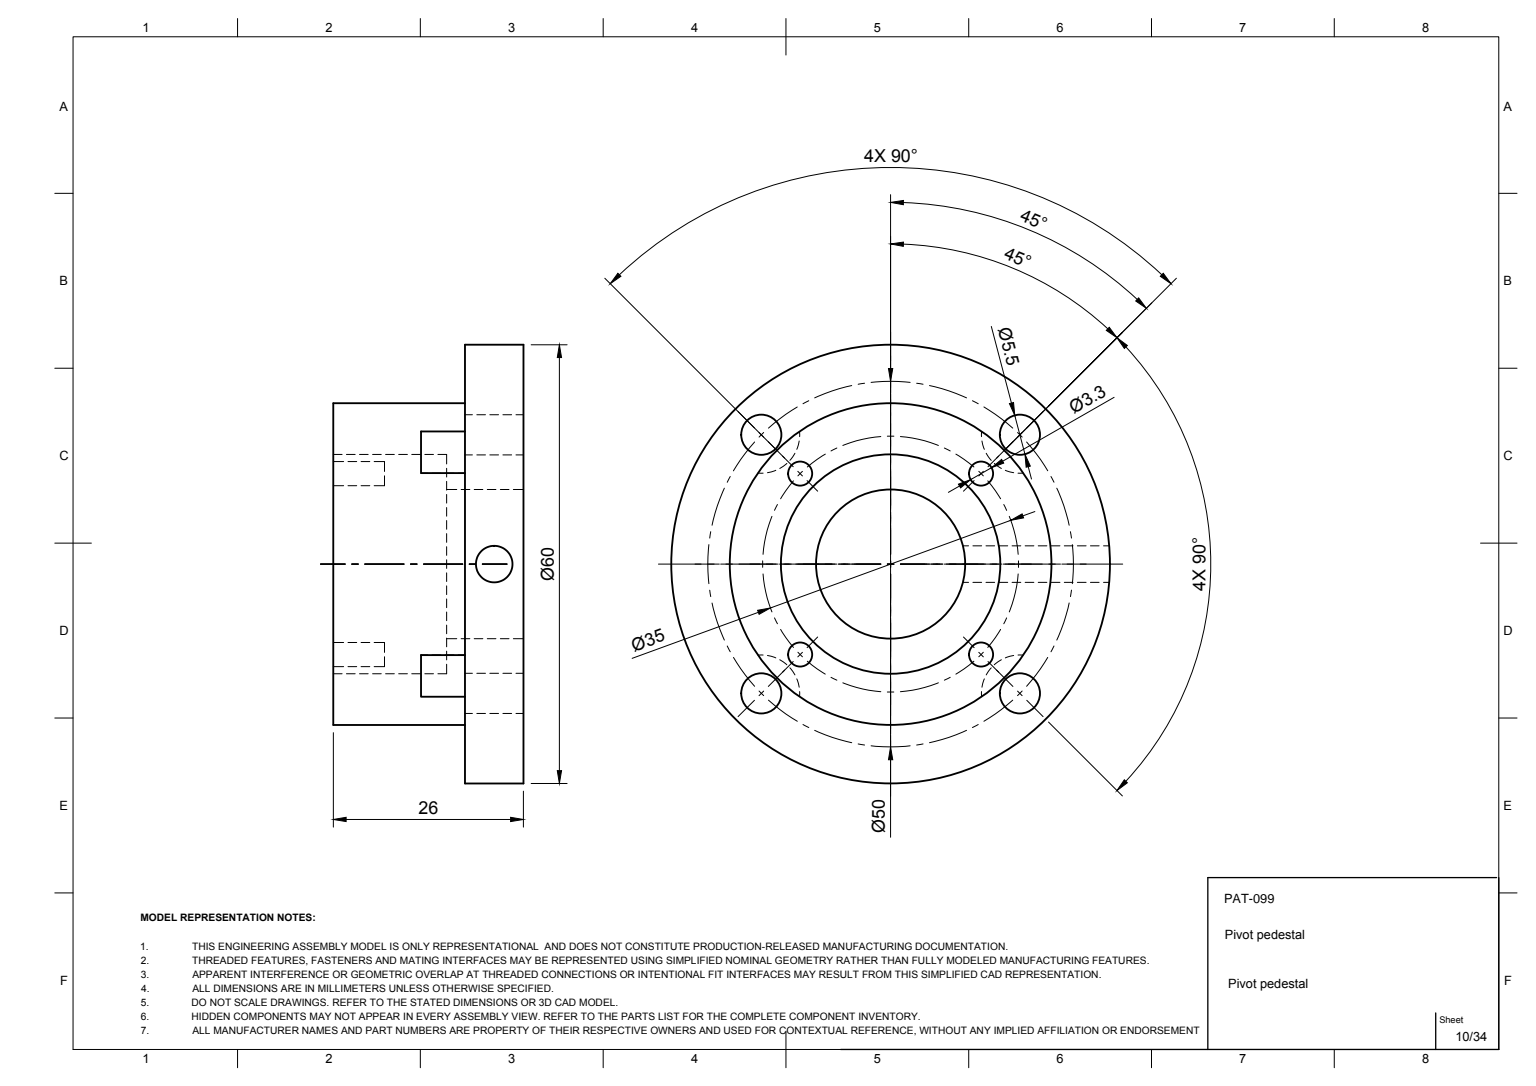
ISO-10303-21;
HEADER;
/* Generated by software containing ST-Developer
 * from STEP Tools, Inc. (www.steptools.com) 
 */

FILE_DESCRIPTION(
/* description */ ('PAT-099'),
/* implementation_level */ '2;1');

FILE_NAME(
/* name */ 'Pivot pedestal.step',
/* time_stamp */ '2026-10-29T17:25:42-07:00',
/* author */ (''),
/* organization */ (''),
/* preprocessor_version */ 'ST-DEVELOPER v20.2',
/* originating_system */ 'Autodesk Translation Framework v15.17.0.0',
/* authorisation */ '');

FILE_SCHEMA (('AUTOMOTIVE_DESIGN { 1 0 10303 214 3 1 1 }'));
ENDSEC;

DATA;
#10=MECHANICAL_DESIGN_GEOMETRIC_PRESENTATION_REPRESENTATION('',(#342),#11035);
#260=B_SPLINE_CURVE_WITH_KNOTS('',3,(#9467,#9468,#9469,#9470,#9471,#9472,
#9473,#9474,#9475,#9476),.UNSPECIFIED.,.F.,.F.,(4,2,2,2,4),(0.,0.0945941824764479,
0.189188364952896,0.283770357603024,0.378352350253152),.UNSPECIFIED.);
#261=B_SPLINE_CURVE_WITH_KNOTS('',3,(#9477,#9478,#9479,#9480,#9481,#9482,
#9483,#9484,#9485,#9486,#9487,#9488,#9489,#9490,#9491,#9492,#9493,#9494,
#9495,#9496,#9497,#9498,#9499,#9500,#9501,#9502),.UNSPECIFIED.,.F.,.F.,
(4,2,2,2,2,2,2,2,2,2,2,2,4),(0.378352350253152,0.47293434290328,0.567516335553408,
0.662110518029855,0.756704700506303,0.851298882982751,0.945893065459199,
1.04047505810933,1.13505705075946,1.22963904340958,1.32422103605971,1.41881521853616,
1.51340940101261),.UNSPECIFIED.);
#262=B_SPLINE_CURVE_WITH_KNOTS('',3,(#9506,#9507,#9508,#9509,#9510,#9511,
#9512,#9513,#9514,#9515,#9516,#9517,#9518,#9519,#9520,#9521,#9522,#9523,
#9524,#9525,#9526,#9527,#9528,#9529,#9530,#9531),.UNSPECIFIED.,.F.,.F.,
(4,2,2,2,2,2,2,2,2,2,2,2,4),(0.,0.0942186410044058,0.188437282008812,0.282655768798837,
0.376874255588861,0.471092742378886,0.565311229168911,0.659529870173317,
0.753748511177723,0.847967152182129,0.942185793186535,1.03640427997656,
1.13062276676658),.UNSPECIFIED.);
#263=B_SPLINE_CURVE_WITH_KNOTS('',3,(#9532,#9533,#9534,#9535,#9536,#9537,
#9538,#9539,#9540,#9541),.UNSPECIFIED.,.F.,.F.,(4,2,2,2,4),(1.13062276676658,
1.22484125355661,1.31905974034663,1.41327838135104,1.50749702235545),
 .UNSPECIFIED.);
#292=SHAPE_REPRESENTATION_RELATIONSHIP('SRR','None',#11160,#317);
#317=ADVANCED_BREP_SHAPE_REPRESENTATION('',(#375),#11010);
#342=STYLED_ITEM('',(#11400),#375);
#375=MANIFOLD_SOLID_BREP('Body1',#4710);
#445=FACE_BOUND('',#1061,.T.);
#446=FACE_BOUND('',#1062,.T.);
#447=FACE_BOUND('',#1063,.T.);
#448=FACE_BOUND('',#1064,.T.);
#449=FACE_BOUND('',#1065,.T.);
#450=FACE_BOUND('',#1072,.T.);
#451=FACE_BOUND('',#1074,.T.);
#452=FACE_BOUND('',#1076,.T.);
#453=FACE_BOUND('',#1078,.T.);
#454=FACE_BOUND('',#1079,.T.);
#455=FACE_BOUND('',#1080,.T.);
#456=FACE_BOUND('',#1081,.T.);
#457=FACE_BOUND('',#1082,.T.);
#458=FACE_BOUND('',#1084,.T.);
#459=FACE_BOUND('',#1085,.T.);
#460=FACE_BOUND('',#1086,.T.);
#461=FACE_BOUND('',#1087,.T.);
#462=FACE_BOUND('',#1088,.T.);
#543=PLANE('',#5153);
#544=PLANE('',#5157);
#545=PLANE('',#5161);
#546=PLANE('',#5165);
#547=PLANE('',#5166);
#548=PLANE('',#5174);
#549=PLANE('',#5179);
#550=PLANE('',#5184);
#551=PLANE('',#5193);
#552=PLANE('',#5210);
#553=PLANE('',#5216);
#554=PLANE('',#5217);
#717=FACE_OUTER_BOUND('',#1042,.T.);
#718=FACE_OUTER_BOUND('',#1043,.T.);
#719=FACE_OUTER_BOUND('',#1044,.T.);
#720=FACE_OUTER_BOUND('',#1045,.T.);
#721=FACE_OUTER_BOUND('',#1046,.T.);
#722=FACE_OUTER_BOUND('',#1047,.T.);
#723=FACE_OUTER_BOUND('',#1048,.T.);
#724=FACE_OUTER_BOUND('',#1049,.T.);
#725=FACE_OUTER_BOUND('',#1050,.T.);
#726=FACE_OUTER_BOUND('',#1051,.T.);
#727=FACE_OUTER_BOUND('',#1052,.T.);
#728=FACE_OUTER_BOUND('',#1053,.T.);
#729=FACE_OUTER_BOUND('',#1054,.T.);
#730=FACE_OUTER_BOUND('',#1055,.T.);
#731=FACE_OUTER_BOUND('',#1056,.T.);
#732=FACE_OUTER_BOUND('',#1057,.T.);
#733=FACE_OUTER_BOUND('',#1058,.T.);
#734=FACE_OUTER_BOUND('',#1059,.T.);
#735=FACE_OUTER_BOUND('',#1060,.T.);
#736=FACE_OUTER_BOUND('',#1066,.T.);
#737=FACE_OUTER_BOUND('',#1067,.T.);
#738=FACE_OUTER_BOUND('',#1068,.T.);
#739=FACE_OUTER_BOUND('',#1069,.T.);
#740=FACE_OUTER_BOUND('',#1070,.T.);
#741=FACE_OUTER_BOUND('',#1071,.T.);
#742=FACE_OUTER_BOUND('',#1073,.T.);
#743=FACE_OUTER_BOUND('',#1075,.T.);
#744=FACE_OUTER_BOUND('',#1077,.T.);
#745=FACE_OUTER_BOUND('',#1083,.T.);
#1042=EDGE_LOOP('',(#3427,#3428,#3429,#3430,#3431,#3432));
#1043=EDGE_LOOP('',(#3433,#3434,#3435,#3436));
#1044=EDGE_LOOP('',(#3437));
#1045=EDGE_LOOP('',(#3438,#3439,#3440,#3441));
#1046=EDGE_LOOP('',(#3442));
#1047=EDGE_LOOP('',(#3443,#3444,#3445,#3446));
#1048=EDGE_LOOP('',(#3447));
#1049=EDGE_LOOP('',(#3448,#3449,#3450,#3451));
#1050=EDGE_LOOP('',(#3452));
#1051=EDGE_LOOP('',(#3453,#3454));
#1052=EDGE_LOOP('',(#3455,#3456,#3457,#3458));
#1053=EDGE_LOOP('',(#3459,#3460,#3461,#3462));
#1054=EDGE_LOOP('',(#3463,#3464));
#1055=EDGE_LOOP('',(#3465,#3466,#3467,#3468));
#1056=EDGE_LOOP('',(#3469,#3470));
#1057=EDGE_LOOP('',(#3471,#3472,#3473,#3474));
#1058=EDGE_LOOP('',(#3475,#3476));
#1059=EDGE_LOOP('',(#3477,#3478,#3479,#3480,#3481,#3482,#3483,#3484,#3485,
#3486,#3487,#3488,#3489,#3490,#3491,#3492,#3493,#3494,#3495,#3496));
#1060=EDGE_LOOP('',(#3497));
#1061=EDGE_LOOP('',(#3498,#3499,#3500,#3501,#3502,#3503,#3504,#3505,#3506));
#1062=EDGE_LOOP('',(#3507));
#1063=EDGE_LOOP('',(#3508));
#1064=EDGE_LOOP('',(#3509));
#1065=EDGE_LOOP('',(#3510));
#1066=EDGE_LOOP('',(#3511,#3512,#3513,#3514));
#1067=EDGE_LOOP('',(#3515,#3516,#3517,#3518));
#1068=EDGE_LOOP('',(#3519,#3520,#3521,#3522));
#1069=EDGE_LOOP('',(#3523,#3524,#3525,#3526));
#1070=EDGE_LOOP('',(#3527,#3528,#3529,#3530));
#1071=EDGE_LOOP('',(#3531));
#1072=EDGE_LOOP('',(#3532));
#1073=EDGE_LOOP('',(#3533,#3534,#3535,#3536));
#1074=EDGE_LOOP('',(#3537,#3538));
#1075=EDGE_LOOP('',(#3539,#3540,#3541,#3542));
#1076=EDGE_LOOP('',(#3543,#3544));
#1077=EDGE_LOOP('',(#3545));
#1078=EDGE_LOOP('',(#3546));
#1079=EDGE_LOOP('',(#3547));
#1080=EDGE_LOOP('',(#3548));
#1081=EDGE_LOOP('',(#3549));
#1082=EDGE_LOOP('',(#3550));
#1083=EDGE_LOOP('',(#3551));
#1084=EDGE_LOOP('',(#3552));
#1085=EDGE_LOOP('',(#3553));
#1086=EDGE_LOOP('',(#3554));
#1087=EDGE_LOOP('',(#3555));
#1088=EDGE_LOOP('',(#3556));
#1404=LINE('',#9504,#1656);
#1405=LINE('',#9546,#1657);
#1406=LINE('',#9553,#1658);
#1407=LINE('',#9560,#1659);
#1408=LINE('',#9567,#1660);
#1409=LINE('',#9577,#1661);
#1410=LINE('',#9580,#1662);
#1411=LINE('',#9584,#1663);
#1412=LINE('',#9588,#1664);
#1413=LINE('',#9595,#1665);
#1414=LINE('',#9599,#1666);
#1415=LINE('',#9606,#1667);
#1416=LINE('',#9610,#1668);
#1417=LINE('',#9618,#1669);
#1418=LINE('',#9638,#1670);
#1419=LINE('',#9642,#1671);
#1420=LINE('',#9646,#1672);
#1421=LINE('',#9650,#1673);
#1422=LINE('',#9655,#1674);
#1423=LINE('',#9662,#1675);
#1424=LINE('',#9666,#1676);
#1656=VECTOR('',#5997,0.25);
#1657=VECTOR('',#6002,0.165);
#1658=VECTOR('',#6011,0.165);
#1659=VECTOR('',#6020,0.165);
#1660=VECTOR('',#6029,0.165);
#1661=VECTOR('',#6042,1.);
#1662=VECTOR('',#6045,1.);
#1663=VECTOR('',#6048,1.);
#1664=VECTOR('',#6051,1.);
#1665=VECTOR('',#6060,1.);
#1666=VECTOR('',#6063,1.);
#1667=VECTOR('',#6072,1.);
#1668=VECTOR('',#6075,1.);
#1669=VECTOR('',#6086,2.2);
#1670=VECTOR('',#6113,0.275);
#1671=VECTOR('',#6118,0.275);
#1672=VECTOR('',#6123,0.275);
#1673=VECTOR('',#6128,0.275);
#1674=VECTOR('',#6133,1.5);
#1675=VECTOR('',#6142,3.);
#1676=VECTOR('',#6147,1.02);
#1915=CIRCLE('',#5151,0.165);
#1916=CIRCLE('',#5152,0.165);
#1917=CIRCLE('',#5155,0.165);
#1918=CIRCLE('',#5156,0.165);
#1919=CIRCLE('',#5159,0.165);
#1920=CIRCLE('',#5160,0.165);
#1921=CIRCLE('',#5163,0.165);
#1922=CIRCLE('',#5164,0.165);
#1923=CIRCLE('',#5167,2.2);
#1924=CIRCLE('',#5168,0.525);
#1925=CIRCLE('',#5170,0.525);
#1926=CIRCLE('',#5172,0.525);
#1927=CIRCLE('',#5173,0.525);
#1928=CIRCLE('',#5175,2.2);
#1929=CIRCLE('',#5177,0.525);
#1930=CIRCLE('',#5178,0.525);
#1931=CIRCLE('',#5180,2.2);
#1932=CIRCLE('',#5182,0.525);
#1933=CIRCLE('',#5183,0.525);
#1934=CIRCLE('',#5185,2.2);
#1935=CIRCLE('',#5187,2.2);
#1936=CIRCLE('',#5188,2.2);
#1937=CIRCLE('',#5189,2.2);
#1938=CIRCLE('',#5190,2.2);
#1939=CIRCLE('',#5191,2.2);
#1940=CIRCLE('',#5192,2.2);
#1941=CIRCLE('',#5194,3.);
#1942=CIRCLE('',#5195,0.275);
#1943=CIRCLE('',#5196,0.275);
#1944=CIRCLE('',#5197,0.275);
#1945=CIRCLE('',#5198,0.275);
#1946=CIRCLE('',#5200,0.275);
#1947=CIRCLE('',#5202,0.275);
#1948=CIRCLE('',#5204,0.275);
#1949=CIRCLE('',#5206,0.275);
#1950=CIRCLE('',#5208,1.5);
#1951=CIRCLE('',#5209,1.5);
#1952=CIRCLE('',#5211,1.02);
#1953=CIRCLE('',#5213,3.);
#1954=CIRCLE('',#5215,1.02);
#2240=VERTEX_POINT('',#9465);
#2241=VERTEX_POINT('',#9466);
#2242=VERTEX_POINT('',#9503);
#2243=VERTEX_POINT('',#9505);
#2244=VERTEX_POINT('',#9543);
#2245=VERTEX_POINT('',#9545);
#2246=VERTEX_POINT('',#9550);
#2247=VERTEX_POINT('',#9552);
#2248=VERTEX_POINT('',#9557);
#2249=VERTEX_POINT('',#9559);
#2250=VERTEX_POINT('',#9564);
#2251=VERTEX_POINT('',#9566);
#2252=VERTEX_POINT('',#9571);
#2253=VERTEX_POINT('',#9572);
#2254=VERTEX_POINT('',#9576);
#2255=VERTEX_POINT('',#9578);
#2256=VERTEX_POINT('',#9582);
#2257=VERTEX_POINT('',#9583);
#2258=VERTEX_POINT('',#9585);
#2259=VERTEX_POINT('',#9587);
#2260=VERTEX_POINT('',#9593);
#2261=VERTEX_POINT('',#9594);
#2262=VERTEX_POINT('',#9596);
#2263=VERTEX_POINT('',#9598);
#2264=VERTEX_POINT('',#9604);
#2265=VERTEX_POINT('',#9605);
#2266=VERTEX_POINT('',#9607);
#2267=VERTEX_POINT('',#9609);
#2268=VERTEX_POINT('',#9615);
#2269=VERTEX_POINT('',#9617);
#2270=VERTEX_POINT('',#9625);
#2271=VERTEX_POINT('',#9627);
#2272=VERTEX_POINT('',#9629);
#2273=VERTEX_POINT('',#9631);
#2274=VERTEX_POINT('',#9633);
#2275=VERTEX_POINT('',#9636);
#2276=VERTEX_POINT('',#9640);
#2277=VERTEX_POINT('',#9644);
#2278=VERTEX_POINT('',#9648);
#2279=VERTEX_POINT('',#9652);
#2280=VERTEX_POINT('',#9654);
#2281=VERTEX_POINT('',#9658);
#2282=VERTEX_POINT('',#9661);
#2283=VERTEX_POINT('',#9665);
#2690=EDGE_CURVE('',#2240,#2241,#260,.T.);
#2691=EDGE_CURVE('',#2241,#2240,#261,.T.);
#2692=EDGE_CURVE('',#2241,#2242,#1404,.T.);
#2693=EDGE_CURVE('',#2243,#2242,#262,.T.);
#2694=EDGE_CURVE('',#2242,#2243,#263,.T.);
#2695=EDGE_CURVE('',#2244,#2244,#1915,.T.);
#2696=EDGE_CURVE('',#2244,#2245,#1405,.T.);
#2697=EDGE_CURVE('',#2245,#2245,#1916,.T.);
#2698=EDGE_CURVE('',#2246,#2246,#1917,.T.);
#2699=EDGE_CURVE('',#2246,#2247,#1406,.T.);
#2700=EDGE_CURVE('',#2247,#2247,#1918,.T.);
#2701=EDGE_CURVE('',#2248,#2248,#1919,.T.);
#2702=EDGE_CURVE('',#2248,#2249,#1407,.T.);
#2703=EDGE_CURVE('',#2249,#2249,#1920,.T.);
#2704=EDGE_CURVE('',#2250,#2250,#1921,.T.);
#2705=EDGE_CURVE('',#2250,#2251,#1408,.T.);
#2706=EDGE_CURVE('',#2251,#2251,#1922,.T.);
#2707=EDGE_CURVE('',#2252,#2253,#1923,.T.);
#2708=EDGE_CURVE('',#2253,#2252,#1924,.T.);
#2709=EDGE_CURVE('',#2254,#2252,#1409,.T.);
#2710=EDGE_CURVE('',#2255,#2254,#1925,.T.);
#2711=EDGE_CURVE('',#2253,#2255,#1410,.T.);
#2712=EDGE_CURVE('',#2256,#2257,#1411,.T.);
#2713=EDGE_CURVE('',#2256,#2258,#1926,.T.);
#2714=EDGE_CURVE('',#2259,#2258,#1412,.T.);
#2715=EDGE_CURVE('',#2257,#2259,#1927,.T.);
#2716=EDGE_CURVE('',#2258,#2256,#1928,.T.);
#2717=EDGE_CURVE('',#2260,#2261,#1413,.T.);
#2718=EDGE_CURVE('',#2260,#2262,#1929,.T.);
#2719=EDGE_CURVE('',#2263,#2262,#1414,.T.);
#2720=EDGE_CURVE('',#2261,#2263,#1930,.T.);
#2721=EDGE_CURVE('',#2262,#2260,#1931,.T.);
#2722=EDGE_CURVE('',#2264,#2265,#1415,.T.);
#2723=EDGE_CURVE('',#2264,#2266,#1932,.T.);
#2724=EDGE_CURVE('',#2267,#2266,#1416,.T.);
#2725=EDGE_CURVE('',#2265,#2267,#1933,.T.);
#2726=EDGE_CURVE('',#2266,#2264,#1934,.T.);
#2727=EDGE_CURVE('',#2268,#2268,#1935,.T.);
#2728=EDGE_CURVE('',#2268,#2269,#1417,.T.);
#2729=EDGE_CURVE('',#2269,#2254,#1936,.T.);
#2730=EDGE_CURVE('',#2255,#2267,#1937,.T.);
#2731=EDGE_CURVE('',#2265,#2263,#1938,.T.);
#2732=EDGE_CURVE('',#2261,#2259,#1939,.T.);
#2733=EDGE_CURVE('',#2257,#2269,#1940,.T.);
#2734=EDGE_CURVE('',#2270,#2270,#1941,.T.);
#2735=EDGE_CURVE('',#2271,#2271,#1942,.T.);
#2736=EDGE_CURVE('',#2272,#2272,#1943,.T.);
#2737=EDGE_CURVE('',#2273,#2273,#1944,.T.);
#2738=EDGE_CURVE('',#2274,#2274,#1945,.T.);
#2739=EDGE_CURVE('',#2275,#2275,#1946,.T.);
#2740=EDGE_CURVE('',#2275,#2271,#1418,.T.);
#2741=EDGE_CURVE('',#2276,#2276,#1947,.T.);
#2742=EDGE_CURVE('',#2276,#2274,#1419,.T.);
#2743=EDGE_CURVE('',#2277,#2277,#1948,.T.);
#2744=EDGE_CURVE('',#2277,#2272,#1420,.T.);
#2745=EDGE_CURVE('',#2278,#2278,#1949,.T.);
#2746=EDGE_CURVE('',#2278,#2273,#1421,.T.);
#2747=EDGE_CURVE('',#2279,#2279,#1950,.T.);
#2748=EDGE_CURVE('',#2279,#2280,#1422,.T.);
#2749=EDGE_CURVE('',#2280,#2280,#1951,.T.);
#2750=EDGE_CURVE('',#2281,#2281,#1952,.T.);
#2751=EDGE_CURVE('',#2270,#2282,#1423,.T.);
#2752=EDGE_CURVE('',#2282,#2282,#1953,.T.);
#2753=EDGE_CURVE('',#2281,#2283,#1424,.T.);
#2754=EDGE_CURVE('',#2283,#2283,#1954,.T.);
#3427=ORIENTED_EDGE('',*,*,#2690,.F.);
#3428=ORIENTED_EDGE('',*,*,#2691,.F.);
#3429=ORIENTED_EDGE('',*,*,#2692,.T.);
#3430=ORIENTED_EDGE('',*,*,#2693,.F.);
#3431=ORIENTED_EDGE('',*,*,#2694,.F.);
#3432=ORIENTED_EDGE('',*,*,#2692,.F.);
#3433=ORIENTED_EDGE('',*,*,#2695,.F.);
#3434=ORIENTED_EDGE('',*,*,#2696,.T.);
#3435=ORIENTED_EDGE('',*,*,#2697,.F.);
#3436=ORIENTED_EDGE('',*,*,#2696,.F.);
#3437=ORIENTED_EDGE('',*,*,#2695,.T.);
#3438=ORIENTED_EDGE('',*,*,#2698,.F.);
#3439=ORIENTED_EDGE('',*,*,#2699,.T.);
#3440=ORIENTED_EDGE('',*,*,#2700,.F.);
#3441=ORIENTED_EDGE('',*,*,#2699,.F.);
#3442=ORIENTED_EDGE('',*,*,#2698,.T.);
#3443=ORIENTED_EDGE('',*,*,#2701,.F.);
#3444=ORIENTED_EDGE('',*,*,#2702,.T.);
#3445=ORIENTED_EDGE('',*,*,#2703,.F.);
#3446=ORIENTED_EDGE('',*,*,#2702,.F.);
#3447=ORIENTED_EDGE('',*,*,#2701,.T.);
#3448=ORIENTED_EDGE('',*,*,#2704,.F.);
#3449=ORIENTED_EDGE('',*,*,#2705,.T.);
#3450=ORIENTED_EDGE('',*,*,#2706,.F.);
#3451=ORIENTED_EDGE('',*,*,#2705,.F.);
#3452=ORIENTED_EDGE('',*,*,#2704,.T.);
#3453=ORIENTED_EDGE('',*,*,#2707,.F.);
#3454=ORIENTED_EDGE('',*,*,#2708,.F.);
#3455=ORIENTED_EDGE('',*,*,#2709,.F.);
#3456=ORIENTED_EDGE('',*,*,#2710,.F.);
#3457=ORIENTED_EDGE('',*,*,#2711,.F.);
#3458=ORIENTED_EDGE('',*,*,#2708,.T.);
#3459=ORIENTED_EDGE('',*,*,#2712,.F.);
#3460=ORIENTED_EDGE('',*,*,#2713,.T.);
#3461=ORIENTED_EDGE('',*,*,#2714,.F.);
#3462=ORIENTED_EDGE('',*,*,#2715,.F.);
#3463=ORIENTED_EDGE('',*,*,#2716,.F.);
#3464=ORIENTED_EDGE('',*,*,#2713,.F.);
#3465=ORIENTED_EDGE('',*,*,#2717,.F.);
#3466=ORIENTED_EDGE('',*,*,#2718,.T.);
#3467=ORIENTED_EDGE('',*,*,#2719,.F.);
#3468=ORIENTED_EDGE('',*,*,#2720,.F.);
#3469=ORIENTED_EDGE('',*,*,#2721,.F.);
#3470=ORIENTED_EDGE('',*,*,#2718,.F.);
#3471=ORIENTED_EDGE('',*,*,#2722,.F.);
#3472=ORIENTED_EDGE('',*,*,#2723,.T.);
#3473=ORIENTED_EDGE('',*,*,#2724,.F.);
#3474=ORIENTED_EDGE('',*,*,#2725,.F.);
#3475=ORIENTED_EDGE('',*,*,#2726,.F.);
#3476=ORIENTED_EDGE('',*,*,#2723,.F.);
#3477=ORIENTED_EDGE('',*,*,#2727,.F.);
#3478=ORIENTED_EDGE('',*,*,#2728,.T.);
#3479=ORIENTED_EDGE('',*,*,#2729,.T.);
#3480=ORIENTED_EDGE('',*,*,#2709,.T.);
#3481=ORIENTED_EDGE('',*,*,#2707,.T.);
#3482=ORIENTED_EDGE('',*,*,#2711,.T.);
#3483=ORIENTED_EDGE('',*,*,#2730,.T.);
#3484=ORIENTED_EDGE('',*,*,#2724,.T.);
#3485=ORIENTED_EDGE('',*,*,#2726,.T.);
#3486=ORIENTED_EDGE('',*,*,#2722,.T.);
#3487=ORIENTED_EDGE('',*,*,#2731,.T.);
#3488=ORIENTED_EDGE('',*,*,#2719,.T.);
#3489=ORIENTED_EDGE('',*,*,#2721,.T.);
#3490=ORIENTED_EDGE('',*,*,#2717,.T.);
#3491=ORIENTED_EDGE('',*,*,#2732,.T.);
#3492=ORIENTED_EDGE('',*,*,#2714,.T.);
#3493=ORIENTED_EDGE('',*,*,#2716,.T.);
#3494=ORIENTED_EDGE('',*,*,#2712,.T.);
#3495=ORIENTED_EDGE('',*,*,#2733,.T.);
#3496=ORIENTED_EDGE('',*,*,#2728,.F.);
#3497=ORIENTED_EDGE('',*,*,#2734,.T.);
#3498=ORIENTED_EDGE('',*,*,#2733,.F.);
#3499=ORIENTED_EDGE('',*,*,#2715,.T.);
#3500=ORIENTED_EDGE('',*,*,#2732,.F.);
#3501=ORIENTED_EDGE('',*,*,#2720,.T.);
#3502=ORIENTED_EDGE('',*,*,#2731,.F.);
#3503=ORIENTED_EDGE('',*,*,#2725,.T.);
#3504=ORIENTED_EDGE('',*,*,#2730,.F.);
#3505=ORIENTED_EDGE('',*,*,#2710,.T.);
#3506=ORIENTED_EDGE('',*,*,#2729,.F.);
#3507=ORIENTED_EDGE('',*,*,#2735,.T.);
#3508=ORIENTED_EDGE('',*,*,#2736,.T.);
#3509=ORIENTED_EDGE('',*,*,#2737,.T.);
#3510=ORIENTED_EDGE('',*,*,#2738,.T.);
#3511=ORIENTED_EDGE('',*,*,#2739,.F.);
#3512=ORIENTED_EDGE('',*,*,#2740,.T.);
#3513=ORIENTED_EDGE('',*,*,#2735,.F.);
#3514=ORIENTED_EDGE('',*,*,#2740,.F.);
#3515=ORIENTED_EDGE('',*,*,#2741,.F.);
#3516=ORIENTED_EDGE('',*,*,#2742,.T.);
#3517=ORIENTED_EDGE('',*,*,#2738,.F.);
#3518=ORIENTED_EDGE('',*,*,#2742,.F.);
#3519=ORIENTED_EDGE('',*,*,#2743,.F.);
#3520=ORIENTED_EDGE('',*,*,#2744,.T.);
#3521=ORIENTED_EDGE('',*,*,#2736,.F.);
#3522=ORIENTED_EDGE('',*,*,#2744,.F.);
#3523=ORIENTED_EDGE('',*,*,#2745,.F.);
#3524=ORIENTED_EDGE('',*,*,#2746,.T.);
#3525=ORIENTED_EDGE('',*,*,#2737,.F.);
#3526=ORIENTED_EDGE('',*,*,#2746,.F.);
#3527=ORIENTED_EDGE('',*,*,#2747,.F.);
#3528=ORIENTED_EDGE('',*,*,#2748,.T.);
#3529=ORIENTED_EDGE('',*,*,#2749,.F.);
#3530=ORIENTED_EDGE('',*,*,#2748,.F.);
#3531=ORIENTED_EDGE('',*,*,#2747,.T.);
#3532=ORIENTED_EDGE('',*,*,#2750,.F.);
#3533=ORIENTED_EDGE('',*,*,#2734,.F.);
#3534=ORIENTED_EDGE('',*,*,#2751,.T.);
#3535=ORIENTED_EDGE('',*,*,#2752,.T.);
#3536=ORIENTED_EDGE('',*,*,#2751,.F.);
#3537=ORIENTED_EDGE('',*,*,#2693,.T.);
#3538=ORIENTED_EDGE('',*,*,#2694,.T.);
#3539=ORIENTED_EDGE('',*,*,#2750,.T.);
#3540=ORIENTED_EDGE('',*,*,#2753,.T.);
#3541=ORIENTED_EDGE('',*,*,#2754,.T.);
#3542=ORIENTED_EDGE('',*,*,#2753,.F.);
#3543=ORIENTED_EDGE('',*,*,#2690,.T.);
#3544=ORIENTED_EDGE('',*,*,#2691,.T.);
#3545=ORIENTED_EDGE('',*,*,#2727,.T.);
#3546=ORIENTED_EDGE('',*,*,#2749,.T.);
#3547=ORIENTED_EDGE('',*,*,#2706,.T.);
#3548=ORIENTED_EDGE('',*,*,#2703,.T.);
#3549=ORIENTED_EDGE('',*,*,#2700,.T.);
#3550=ORIENTED_EDGE('',*,*,#2697,.T.);
#3551=ORIENTED_EDGE('',*,*,#2752,.F.);
#3552=ORIENTED_EDGE('',*,*,#2754,.F.);
#3553=ORIENTED_EDGE('',*,*,#2745,.T.);
#3554=ORIENTED_EDGE('',*,*,#2743,.T.);
#3555=ORIENTED_EDGE('',*,*,#2741,.T.);
#3556=ORIENTED_EDGE('',*,*,#2739,.T.);
#4346=CYLINDRICAL_SURFACE('',#5149,0.25);
#4347=CYLINDRICAL_SURFACE('',#5150,0.165);
#4348=CYLINDRICAL_SURFACE('',#5154,0.165);
#4349=CYLINDRICAL_SURFACE('',#5158,0.165);
#4350=CYLINDRICAL_SURFACE('',#5162,0.165);
#4351=CYLINDRICAL_SURFACE('',#5169,0.525);
#4352=CYLINDRICAL_SURFACE('',#5171,0.525);
#4353=CYLINDRICAL_SURFACE('',#5176,0.525);
#4354=CYLINDRICAL_SURFACE('',#5181,0.525);
#4355=CYLINDRICAL_SURFACE('',#5186,2.2);
#4356=CYLINDRICAL_SURFACE('',#5199,0.275);
#4357=CYLINDRICAL_SURFACE('',#5201,0.275);
#4358=CYLINDRICAL_SURFACE('',#5203,0.275);
#4359=CYLINDRICAL_SURFACE('',#5205,0.275);
#4360=CYLINDRICAL_SURFACE('',#5207,1.5);
#4361=CYLINDRICAL_SURFACE('',#5212,3.);
#4362=CYLINDRICAL_SURFACE('',#5214,1.02);
#4482=ADVANCED_FACE('',(#717),#4346,.F.);
#4483=ADVANCED_FACE('',(#718),#4347,.F.);
#4484=ADVANCED_FACE('',(#719),#543,.T.);
#4485=ADVANCED_FACE('',(#720),#4348,.F.);
#4486=ADVANCED_FACE('',(#721),#544,.T.);
#4487=ADVANCED_FACE('',(#722),#4349,.F.);
#4488=ADVANCED_FACE('',(#723),#545,.T.);
#4489=ADVANCED_FACE('',(#724),#4350,.F.);
#4490=ADVANCED_FACE('',(#725),#546,.T.);
#4491=ADVANCED_FACE('',(#726),#547,.F.);
#4492=ADVANCED_FACE('',(#727),#4351,.F.);
#4493=ADVANCED_FACE('',(#728),#4352,.F.);
#4494=ADVANCED_FACE('',(#729),#548,.F.);
#4495=ADVANCED_FACE('',(#730),#4353,.F.);
#4496=ADVANCED_FACE('',(#731),#549,.F.);
#4497=ADVANCED_FACE('',(#732),#4354,.F.);
#4498=ADVANCED_FACE('',(#733),#550,.F.);
#4499=ADVANCED_FACE('',(#734),#4355,.T.);
#4500=ADVANCED_FACE('',(#735,#445,#446,#447,#448,#449),#551,.T.);
#4501=ADVANCED_FACE('',(#736),#4356,.F.);
#4502=ADVANCED_FACE('',(#737),#4357,.F.);
#4503=ADVANCED_FACE('',(#738),#4358,.F.);
#4504=ADVANCED_FACE('',(#739),#4359,.F.);
#4505=ADVANCED_FACE('',(#740),#4360,.F.);
#4506=ADVANCED_FACE('',(#741,#450),#552,.T.);
#4507=ADVANCED_FACE('',(#742,#451),#4361,.T.);
#4508=ADVANCED_FACE('',(#743,#452),#4362,.F.);
#4509=ADVANCED_FACE('',(#744,#453,#454,#455,#456,#457),#553,.T.);
#4510=ADVANCED_FACE('',(#745,#458,#459,#460,#461,#462),#554,.F.);
#4710=CLOSED_SHELL('',(#4482,#4483,#4484,#4485,#4486,#4487,#4488,#4489,
#4490,#4491,#4492,#4493,#4494,#4495,#4496,#4497,#4498,#4499,#4500,#4501,
#4502,#4503,#4504,#4505,#4506,#4507,#4508,#4509,#4510));
#5148=AXIS2_PLACEMENT_3D('',#9463,#5993,#5994);
#5149=AXIS2_PLACEMENT_3D('',#9464,#5995,#5996);
#5150=AXIS2_PLACEMENT_3D('',#9542,#5998,#5999);
#5151=AXIS2_PLACEMENT_3D('',#9544,#6000,#6001);
#5152=AXIS2_PLACEMENT_3D('',#9547,#6003,#6004);
#5153=AXIS2_PLACEMENT_3D('',#9548,#6005,#6006);
#5154=AXIS2_PLACEMENT_3D('',#9549,#6007,#6008);
#5155=AXIS2_PLACEMENT_3D('',#9551,#6009,#6010);
#5156=AXIS2_PLACEMENT_3D('',#9554,#6012,#6013);
#5157=AXIS2_PLACEMENT_3D('',#9555,#6014,#6015);
#5158=AXIS2_PLACEMENT_3D('',#9556,#6016,#6017);
#5159=AXIS2_PLACEMENT_3D('',#9558,#6018,#6019);
#5160=AXIS2_PLACEMENT_3D('',#9561,#6021,#6022);
#5161=AXIS2_PLACEMENT_3D('',#9562,#6023,#6024);
#5162=AXIS2_PLACEMENT_3D('',#9563,#6025,#6026);
#5163=AXIS2_PLACEMENT_3D('',#9565,#6027,#6028);
#5164=AXIS2_PLACEMENT_3D('',#9568,#6030,#6031);
#5165=AXIS2_PLACEMENT_3D('',#9569,#6032,#6033);
#5166=AXIS2_PLACEMENT_3D('',#9570,#6034,#6035);
#5167=AXIS2_PLACEMENT_3D('',#9573,#6036,#6037);
#5168=AXIS2_PLACEMENT_3D('',#9574,#6038,#6039);
#5169=AXIS2_PLACEMENT_3D('',#9575,#6040,#6041);
#5170=AXIS2_PLACEMENT_3D('',#9579,#6043,#6044);
#5171=AXIS2_PLACEMENT_3D('',#9581,#6046,#6047);
#5172=AXIS2_PLACEMENT_3D('',#9586,#6049,#6050);
#5173=AXIS2_PLACEMENT_3D('',#9589,#6052,#6053);
#5174=AXIS2_PLACEMENT_3D('',#9590,#6054,#6055);
#5175=AXIS2_PLACEMENT_3D('',#9591,#6056,#6057);
#5176=AXIS2_PLACEMENT_3D('',#9592,#6058,#6059);
#5177=AXIS2_PLACEMENT_3D('',#9597,#6061,#6062);
#5178=AXIS2_PLACEMENT_3D('',#9600,#6064,#6065);
#5179=AXIS2_PLACEMENT_3D('',#9601,#6066,#6067);
#5180=AXIS2_PLACEMENT_3D('',#9602,#6068,#6069);
#5181=AXIS2_PLACEMENT_3D('',#9603,#6070,#6071);
#5182=AXIS2_PLACEMENT_3D('',#9608,#6073,#6074);
#5183=AXIS2_PLACEMENT_3D('',#9611,#6076,#6077);
#5184=AXIS2_PLACEMENT_3D('',#9612,#6078,#6079);
#5185=AXIS2_PLACEMENT_3D('',#9613,#6080,#6081);
#5186=AXIS2_PLACEMENT_3D('',#9614,#6082,#6083);
#5187=AXIS2_PLACEMENT_3D('',#9616,#6084,#6085);
#5188=AXIS2_PLACEMENT_3D('',#9619,#6087,#6088);
#5189=AXIS2_PLACEMENT_3D('',#9620,#6089,#6090);
#5190=AXIS2_PLACEMENT_3D('',#9621,#6091,#6092);
#5191=AXIS2_PLACEMENT_3D('',#9622,#6093,#6094);
#5192=AXIS2_PLACEMENT_3D('',#9623,#6095,#6096);
#5193=AXIS2_PLACEMENT_3D('',#9624,#6097,#6098);
#5194=AXIS2_PLACEMENT_3D('',#9626,#6099,#6100);
#5195=AXIS2_PLACEMENT_3D('',#9628,#6101,#6102);
#5196=AXIS2_PLACEMENT_3D('',#9630,#6103,#6104);
#5197=AXIS2_PLACEMENT_3D('',#9632,#6105,#6106);
#5198=AXIS2_PLACEMENT_3D('',#9634,#6107,#6108);
#5199=AXIS2_PLACEMENT_3D('',#9635,#6109,#6110);
#5200=AXIS2_PLACEMENT_3D('',#9637,#6111,#6112);
#5201=AXIS2_PLACEMENT_3D('',#9639,#6114,#6115);
#5202=AXIS2_PLACEMENT_3D('',#9641,#6116,#6117);
#5203=AXIS2_PLACEMENT_3D('',#9643,#6119,#6120);
#5204=AXIS2_PLACEMENT_3D('',#9645,#6121,#6122);
#5205=AXIS2_PLACEMENT_3D('',#9647,#6124,#6125);
#5206=AXIS2_PLACEMENT_3D('',#9649,#6126,#6127);
#5207=AXIS2_PLACEMENT_3D('',#9651,#6129,#6130);
#5208=AXIS2_PLACEMENT_3D('',#9653,#6131,#6132);
#5209=AXIS2_PLACEMENT_3D('',#9656,#6134,#6135);
#5210=AXIS2_PLACEMENT_3D('',#9657,#6136,#6137);
#5211=AXIS2_PLACEMENT_3D('',#9659,#6138,#6139);
#5212=AXIS2_PLACEMENT_3D('',#9660,#6140,#6141);
#5213=AXIS2_PLACEMENT_3D('',#9663,#6143,#6144);
#5214=AXIS2_PLACEMENT_3D('',#9664,#6145,#6146);
#5215=AXIS2_PLACEMENT_3D('',#9667,#6148,#6149);
#5216=AXIS2_PLACEMENT_3D('',#9668,#6150,#6151);
#5217=AXIS2_PLACEMENT_3D('',#9669,#6152,#6153);
#5993=DIRECTION('axis',(0.,0.,1.));
#5994=DIRECTION('refdir',(1.,0.,0.));
#5995=DIRECTION('center_axis',(1.,0.,0.));
#5996=DIRECTION('ref_axis',(0.,0.,-1.));
#5997=DIRECTION('',(1.,0.,0.));
#5998=DIRECTION('center_axis',(0.,0.,1.));
#5999=DIRECTION('ref_axis',(1.,0.,0.));
#6000=DIRECTION('center_axis',(0.,0.,1.));
#6001=DIRECTION('ref_axis',(1.,0.,0.));
#6002=DIRECTION('',(0.,0.,1.));
#6003=DIRECTION('center_axis',(0.,0.,-1.));
#6004=DIRECTION('ref_axis',(1.,0.,0.));
#6005=DIRECTION('center_axis',(0.,0.,1.));
#6006=DIRECTION('ref_axis',(1.,0.,0.));
#6007=DIRECTION('center_axis',(0.,0.,1.));
#6008=DIRECTION('ref_axis',(1.,0.,0.));
#6009=DIRECTION('center_axis',(0.,0.,1.));
#6010=DIRECTION('ref_axis',(1.,0.,0.));
#6011=DIRECTION('',(0.,0.,1.));
#6012=DIRECTION('center_axis',(0.,0.,-1.));
#6013=DIRECTION('ref_axis',(1.,0.,0.));
#6014=DIRECTION('center_axis',(0.,0.,1.));
#6015=DIRECTION('ref_axis',(1.,0.,0.));
#6016=DIRECTION('center_axis',(0.,0.,1.));
#6017=DIRECTION('ref_axis',(1.,0.,0.));
#6018=DIRECTION('center_axis',(0.,0.,1.));
#6019=DIRECTION('ref_axis',(1.,0.,0.));
#6020=DIRECTION('',(0.,0.,1.));
#6021=DIRECTION('center_axis',(0.,0.,-1.));
#6022=DIRECTION('ref_axis',(1.,0.,0.));
#6023=DIRECTION('center_axis',(0.,0.,1.));
#6024=DIRECTION('ref_axis',(1.,0.,0.));
#6025=DIRECTION('center_axis',(0.,0.,1.));
#6026=DIRECTION('ref_axis',(1.,0.,0.));
#6027=DIRECTION('center_axis',(0.,0.,1.));
#6028=DIRECTION('ref_axis',(1.,0.,0.));
#6029=DIRECTION('',(0.,0.,1.));
#6030=DIRECTION('center_axis',(0.,0.,-1.));
#6031=DIRECTION('ref_axis',(1.,0.,0.));
#6032=DIRECTION('center_axis',(0.,0.,1.));
#6033=DIRECTION('ref_axis',(1.,0.,0.));
#6034=DIRECTION('center_axis',(0.,0.,1.));
#6035=DIRECTION('ref_axis',(1.,0.,0.));
#6036=DIRECTION('center_axis',(0.,0.,1.));
#6037=DIRECTION('ref_axis',(1.,0.,0.));
#6038=DIRECTION('center_axis',(0.,0.,1.));
#6039=DIRECTION('ref_axis',(1.,0.,0.));
#6040=DIRECTION('center_axis',(0.,0.,1.));
#6041=DIRECTION('ref_axis',(1.,0.,0.));
#6042=DIRECTION('',(0.,0.,1.));
#6043=DIRECTION('center_axis',(0.,0.,1.));
#6044=DIRECTION('ref_axis',(1.,0.,0.));
#6045=DIRECTION('',(0.,0.,-1.));
#6046=DIRECTION('center_axis',(0.,0.,1.));
#6047=DIRECTION('ref_axis',(1.,0.,0.));
#6048=DIRECTION('',(0.,0.,-1.));
#6049=DIRECTION('center_axis',(0.,0.,1.));
#6050=DIRECTION('ref_axis',(1.,0.,0.));
#6051=DIRECTION('',(0.,0.,1.));
#6052=DIRECTION('center_axis',(0.,0.,1.));
#6053=DIRECTION('ref_axis',(1.,0.,0.));
#6054=DIRECTION('center_axis',(0.,0.,1.));
#6055=DIRECTION('ref_axis',(1.,0.,0.));
#6056=DIRECTION('center_axis',(0.,0.,1.));
#6057=DIRECTION('ref_axis',(1.,0.,0.));
#6058=DIRECTION('center_axis',(0.,0.,1.));
#6059=DIRECTION('ref_axis',(-0.707106781186548,-0.707106781186547,0.));
#6060=DIRECTION('',(0.,0.,-1.));
#6061=DIRECTION('center_axis',(0.,0.,1.));
#6062=DIRECTION('ref_axis',(1.,0.,0.));
#6063=DIRECTION('',(0.,0.,1.));
#6064=DIRECTION('center_axis',(0.,0.,1.));
#6065=DIRECTION('ref_axis',(1.,0.,0.));
#6066=DIRECTION('center_axis',(0.,0.,1.));
#6067=DIRECTION('ref_axis',(1.,0.,0.));
#6068=DIRECTION('center_axis',(0.,0.,1.));
#6069=DIRECTION('ref_axis',(1.,0.,0.));
#6070=DIRECTION('center_axis',(0.,0.,1.));
#6071=DIRECTION('ref_axis',(-0.707106781186547,0.707106781186548,0.));
#6072=DIRECTION('',(0.,0.,-1.));
#6073=DIRECTION('center_axis',(0.,0.,1.));
#6074=DIRECTION('ref_axis',(1.,0.,0.));
#6075=DIRECTION('',(0.,0.,1.));
#6076=DIRECTION('center_axis',(0.,0.,1.));
#6077=DIRECTION('ref_axis',(1.,0.,0.));
#6078=DIRECTION('center_axis',(0.,0.,1.));
#6079=DIRECTION('ref_axis',(1.,0.,0.));
#6080=DIRECTION('center_axis',(0.,0.,1.));
#6081=DIRECTION('ref_axis',(1.,0.,0.));
#6082=DIRECTION('center_axis',(0.,0.,1.));
#6083=DIRECTION('ref_axis',(1.,0.,0.));
#6084=DIRECTION('center_axis',(0.,0.,1.));
#6085=DIRECTION('ref_axis',(1.,0.,0.));
#6086=DIRECTION('',(0.,0.,-1.));
#6087=DIRECTION('center_axis',(0.,0.,1.));
#6088=DIRECTION('ref_axis',(1.,0.,0.));
#6089=DIRECTION('center_axis',(0.,0.,1.));
#6090=DIRECTION('ref_axis',(1.,0.,0.));
#6091=DIRECTION('center_axis',(0.,0.,1.));
#6092=DIRECTION('ref_axis',(1.,0.,0.));
#6093=DIRECTION('center_axis',(0.,0.,1.));
#6094=DIRECTION('ref_axis',(1.,0.,0.));
#6095=DIRECTION('center_axis',(0.,0.,1.));
#6096=DIRECTION('ref_axis',(1.,0.,0.));
#6097=DIRECTION('center_axis',(0.,0.,1.));
#6098=DIRECTION('ref_axis',(1.,0.,0.));
#6099=DIRECTION('center_axis',(0.,0.,1.));
#6100=DIRECTION('ref_axis',(1.,0.,0.));
#6101=DIRECTION('center_axis',(0.,0.,-1.));
#6102=DIRECTION('ref_axis',(1.,0.,0.));
#6103=DIRECTION('center_axis',(0.,0.,-1.));
#6104=DIRECTION('ref_axis',(1.,0.,0.));
#6105=DIRECTION('center_axis',(0.,0.,-1.));
#6106=DIRECTION('ref_axis',(1.,0.,0.));
#6107=DIRECTION('center_axis',(0.,0.,-1.));
#6108=DIRECTION('ref_axis',(1.,0.,0.));
#6109=DIRECTION('center_axis',(0.,0.,1.));
#6110=DIRECTION('ref_axis',(1.,0.,0.));
#6111=DIRECTION('center_axis',(0.,0.,1.));
#6112=DIRECTION('ref_axis',(1.,0.,0.));
#6113=DIRECTION('',(0.,0.,1.));
#6114=DIRECTION('center_axis',(0.,0.,1.));
#6115=DIRECTION('ref_axis',(1.,0.,0.));
#6116=DIRECTION('center_axis',(0.,0.,1.));
#6117=DIRECTION('ref_axis',(1.,0.,0.));
#6118=DIRECTION('',(0.,0.,1.));
#6119=DIRECTION('center_axis',(0.,0.,1.));
#6120=DIRECTION('ref_axis',(1.,0.,0.));
#6121=DIRECTION('center_axis',(0.,0.,1.));
#6122=DIRECTION('ref_axis',(1.,0.,0.));
#6123=DIRECTION('',(0.,0.,1.));
#6124=DIRECTION('center_axis',(0.,0.,1.));
#6125=DIRECTION('ref_axis',(1.,0.,0.));
#6126=DIRECTION('center_axis',(0.,0.,1.));
#6127=DIRECTION('ref_axis',(1.,0.,0.));
#6128=DIRECTION('',(0.,0.,1.));
#6129=DIRECTION('center_axis',(0.,0.,1.));
#6130=DIRECTION('ref_axis',(1.,0.,0.));
#6131=DIRECTION('center_axis',(0.,0.,1.));
#6132=DIRECTION('ref_axis',(1.,0.,0.));
#6133=DIRECTION('',(0.,0.,1.));
#6134=DIRECTION('center_axis',(0.,0.,-1.));
#6135=DIRECTION('ref_axis',(1.,0.,0.));
#6136=DIRECTION('center_axis',(0.,0.,1.));
#6137=DIRECTION('ref_axis',(1.,0.,0.));
#6138=DIRECTION('center_axis',(0.,0.,1.));
#6139=DIRECTION('ref_axis',(1.,0.,0.));
#6140=DIRECTION('center_axis',(0.,0.,1.));
#6141=DIRECTION('ref_axis',(1.,0.,0.));
#6142=DIRECTION('',(0.,0.,-1.));
#6143=DIRECTION('center_axis',(0.,0.,1.));
#6144=DIRECTION('ref_axis',(1.,0.,0.));
#6145=DIRECTION('center_axis',(0.,0.,1.));
#6146=DIRECTION('ref_axis',(1.,0.,0.));
#6147=DIRECTION('',(0.,0.,-1.));
#6148=DIRECTION('center_axis',(0.,0.,-1.));
#6149=DIRECTION('ref_axis',(1.,0.,0.));
#6150=DIRECTION('center_axis',(0.,0.,1.));
#6151=DIRECTION('ref_axis',(1.,0.,0.));
#6152=DIRECTION('center_axis',(0.,0.,1.));
#6153=DIRECTION('ref_axis',(1.,0.,0.));
#9463=CARTESIAN_POINT('',(0.,0.,0.));
#9464=CARTESIAN_POINT('Origin',(0.9,0.,1.4));
#9465=CARTESIAN_POINT('',(0.988888264668966,0.25,1.4));
#9466=CARTESIAN_POINT('',(1.02,-1.18386380373883E-17,1.65));
#9467=CARTESIAN_POINT('Ctrl Pts',(0.988888264668966,0.25,1.4));
#9468=CARTESIAN_POINT('Ctrl Pts',(0.988888264668966,0.25,1.43153139415882));
#9469=CARTESIAN_POINT('Ctrl Pts',(0.990553370646674,0.243672048431404,1.46507214966317));
#9470=CARTESIAN_POINT('Ctrl Pts',(0.996491737296663,0.218119830014375,1.52662620974954));
#9471=CARTESIAN_POINT('Ctrl Pts',(1.00067109353237,0.198902128206072,1.5546512623872));
#9472=CARTESIAN_POINT('Ctrl Pts',(1.00845756932386,0.154654113568716,1.59889927702456));
#9473=CARTESIAN_POINT('Ctrl Pts',(1.01258144235289,0.126627870945253,1.61811920309393));
#9474=CARTESIAN_POINT('Ctrl Pts',(1.0183917429657,0.065069600391363,1.64367304400768));
#9475=CARTESIAN_POINT('Ctrl Pts',(1.02,0.031527330883376,1.65));
#9476=CARTESIAN_POINT('Ctrl Pts',(1.02,2.77555756156289E-17,1.65));
#9477=CARTESIAN_POINT('Ctrl Pts',(1.02,6.93889390390723E-18,1.65));
#9478=CARTESIAN_POINT('Ctrl Pts',(1.02,-0.031527330883376,1.65));
#9479=CARTESIAN_POINT('Ctrl Pts',(1.0183917429657,-0.065069600391363,1.64367304400768));
#9480=CARTESIAN_POINT('Ctrl Pts',(1.01258144235289,-0.126627870945253,1.61811920309393));
#9481=CARTESIAN_POINT('Ctrl Pts',(1.00845756932386,-0.154654113568716,1.59889927702456));
#9482=CARTESIAN_POINT('Ctrl Pts',(1.00067109353237,-0.198902128206072,1.5546512623872));
#9483=CARTESIAN_POINT('Ctrl Pts',(0.996491737296663,-0.218119830014375,
1.52662620974954));
#9484=CARTESIAN_POINT('Ctrl Pts',(0.990553370646674,-0.243672048431404,
1.46507214966317));
#9485=CARTESIAN_POINT('Ctrl Pts',(0.988888264668967,-0.25,1.43153139415882));
#9486=CARTESIAN_POINT('Ctrl Pts',(0.988888264668967,-0.25,1.36846860584118));
#9487=CARTESIAN_POINT('Ctrl Pts',(0.990553370646674,-0.243672048431404,
1.33492785033683));
#9488=CARTESIAN_POINT('Ctrl Pts',(0.996491737296663,-0.218119830014375,
1.27337379025046));
#9489=CARTESIAN_POINT('Ctrl Pts',(1.00067109353237,-0.198902128206072,1.2453487376128));
#9490=CARTESIAN_POINT('Ctrl Pts',(1.00845756932386,-0.154654113568716,1.20110072297544));
#9491=CARTESIAN_POINT('Ctrl Pts',(1.01258144235289,-0.126627870945254,1.18188079690607));
#9492=CARTESIAN_POINT('Ctrl Pts',(1.0183917429657,-0.0650696003913633,1.15632695599232));
#9493=CARTESIAN_POINT('Ctrl Pts',(1.02,-0.0315273308833761,1.15));
#9494=CARTESIAN_POINT('Ctrl Pts',(1.02,0.0315273308833759,1.15));
#9495=CARTESIAN_POINT('Ctrl Pts',(1.0183917429657,0.065069600391363,1.15632695599232));
#9496=CARTESIAN_POINT('Ctrl Pts',(1.01258144235289,0.126627870945253,1.18188079690607));
#9497=CARTESIAN_POINT('Ctrl Pts',(1.00845756932386,0.154654113568716,1.20110072297544));
#9498=CARTESIAN_POINT('Ctrl Pts',(1.00067109353237,0.198902128206072,1.2453487376128));
#9499=CARTESIAN_POINT('Ctrl Pts',(0.996491737296663,0.218119830014375,1.27337379025046));
#9500=CARTESIAN_POINT('Ctrl Pts',(0.990553370646674,0.243672048431404,1.33492785033683));
#9501=CARTESIAN_POINT('Ctrl Pts',(0.988888264668967,0.25,1.36846860584118));
#9502=CARTESIAN_POINT('Ctrl Pts',(0.988888264668967,0.25,1.4));
#9503=CARTESIAN_POINT('',(3.,-3.06161699786838E-17,1.65));
#9504=CARTESIAN_POINT('',(0.9,-3.06161699786838E-17,1.65));
#9505=CARTESIAN_POINT('',(2.98956518577535,0.25,1.4));
#9506=CARTESIAN_POINT('Ctrl Pts',(2.98956518577535,0.25,1.4));
#9507=CARTESIAN_POINT('Ctrl Pts',(2.98956518577535,0.25,1.36859378633186));
#9508=CARTESIAN_POINT('Ctrl Pts',(2.99011104995181,0.24372047740942,1.33510417960069));
#9509=CARTESIAN_POINT('Ctrl Pts',(2.99208145165098,0.218202539734559,1.27351367328886));
#9510=CARTESIAN_POINT('Ctrl Pts',(2.99347740802958,0.198964922639276,1.245411532046));
#9511=CARTESIAN_POINT('Ctrl Pts',(2.99609686518216,0.154588504271054,1.20103511367778));
#9512=CARTESIAN_POINT('Ctrl Pts',(2.99749070376198,0.126486346986081,1.18179746841036));
#9513=CARTESIAN_POINT('Ctrl Pts',(2.99945625936844,0.0648957875009219,1.15627950921557));
#9514=CARTESIAN_POINT('Ctrl Pts',(3.,0.0314061622633416,1.15));
#9515=CARTESIAN_POINT('Ctrl Pts',(3.,-0.0314061622633416,1.15));
#9516=CARTESIAN_POINT('Ctrl Pts',(2.99945625936844,-0.0648957875009221,
1.15627950921557));
#9517=CARTESIAN_POINT('Ctrl Pts',(2.99749070376198,-0.126486346986081,1.18179746841036));
#9518=CARTESIAN_POINT('Ctrl Pts',(2.99609686518216,-0.154588504271054,1.20103511367778));
#9519=CARTESIAN_POINT('Ctrl Pts',(2.99347740802958,-0.198964922639276,1.245411532046));
#9520=CARTESIAN_POINT('Ctrl Pts',(2.99208145165098,-0.218202539734559,1.27351367328886));
#9521=CARTESIAN_POINT('Ctrl Pts',(2.99011104995181,-0.24372047740942,1.33510417960069));
#9522=CARTESIAN_POINT('Ctrl Pts',(2.98956518577535,-0.25,1.36859378633186));
#9523=CARTESIAN_POINT('Ctrl Pts',(2.98956518577535,-0.25,1.43140621366814));
#9524=CARTESIAN_POINT('Ctrl Pts',(2.99011104995181,-0.24372047740942,1.4648958203993));
#9525=CARTESIAN_POINT('Ctrl Pts',(2.99208145165098,-0.21820253973456,1.52648632671114));
#9526=CARTESIAN_POINT('Ctrl Pts',(2.99347740802958,-0.198964922639276,1.554588467954));
#9527=CARTESIAN_POINT('Ctrl Pts',(2.99609686518216,-0.154588504271054,1.59896488632222));
#9528=CARTESIAN_POINT('Ctrl Pts',(2.99749070376198,-0.126486346986082,1.61820253158964));
#9529=CARTESIAN_POINT('Ctrl Pts',(2.99945625936844,-0.0648957875009221,
1.64372049078443));
#9530=CARTESIAN_POINT('Ctrl Pts',(3.,-0.0314061622633417,1.65));
#9531=CARTESIAN_POINT('Ctrl Pts',(3.,-5.55111512312578E-17,1.65));
#9532=CARTESIAN_POINT('Ctrl Pts',(3.,-2.08166817117217E-17,1.65));
#9533=CARTESIAN_POINT('Ctrl Pts',(3.,0.0314061622633416,1.65));
#9534=CARTESIAN_POINT('Ctrl Pts',(2.99945625936844,0.0648957875009221,1.64372049078443));
#9535=CARTESIAN_POINT('Ctrl Pts',(2.99749070376198,0.126486346986081,1.61820253158964));
#9536=CARTESIAN_POINT('Ctrl Pts',(2.99609686518216,0.154588504271054,1.59896488632222));
#9537=CARTESIAN_POINT('Ctrl Pts',(2.99347740802958,0.198964922639276,1.554588467954));
#9538=CARTESIAN_POINT('Ctrl Pts',(2.99208145165098,0.218202539734559,1.52648632671114));
#9539=CARTESIAN_POINT('Ctrl Pts',(2.99011104995181,0.24372047740942,1.46489582039931));
#9540=CARTESIAN_POINT('Ctrl Pts',(2.98956518577535,0.25,1.43140621366814));
#9541=CARTESIAN_POINT('Ctrl Pts',(2.98956518577535,0.25,1.4));
#9542=CARTESIAN_POINT('Origin',(-1.23743686707646,-1.23743686707646,2.9));
#9543=CARTESIAN_POINT('',(-1.40243686707646,-1.23743686707646,2.9));
#9544=CARTESIAN_POINT('Origin',(-1.23743686707646,-1.23743686707646,2.9));
#9545=CARTESIAN_POINT('',(-1.40243686707646,-1.23743686707646,3.6));
#9546=CARTESIAN_POINT('',(-1.40243686707646,-1.23743686707646,2.9));
#9547=CARTESIAN_POINT('Origin',(-1.23743686707646,-1.23743686707646,3.6));
#9548=CARTESIAN_POINT('Origin',(-1.23743686707646,-1.23743686707646,2.9));
#9549=CARTESIAN_POINT('Origin',(-1.23743686707646,1.23743686707646,2.9));
#9550=CARTESIAN_POINT('',(-1.40243686707646,1.23743686707646,2.9));
#9551=CARTESIAN_POINT('Origin',(-1.23743686707646,1.23743686707646,2.9));
#9552=CARTESIAN_POINT('',(-1.40243686707646,1.23743686707646,3.6));
#9553=CARTESIAN_POINT('',(-1.40243686707646,1.23743686707646,2.9));
#9554=CARTESIAN_POINT('Origin',(-1.23743686707646,1.23743686707646,3.6));
#9555=CARTESIAN_POINT('Origin',(-1.23743686707646,1.23743686707646,2.9));
#9556=CARTESIAN_POINT('Origin',(1.23743686707646,1.23743686707646,2.9));
#9557=CARTESIAN_POINT('',(1.07243686707646,1.23743686707646,2.9));
#9558=CARTESIAN_POINT('Origin',(1.23743686707646,1.23743686707646,2.9));
#9559=CARTESIAN_POINT('',(1.07243686707646,1.23743686707646,3.6));
#9560=CARTESIAN_POINT('',(1.07243686707646,1.23743686707646,2.9));
#9561=CARTESIAN_POINT('Origin',(1.23743686707646,1.23743686707646,3.6));
#9562=CARTESIAN_POINT('Origin',(1.23743686707646,1.23743686707646,2.9));
#9563=CARTESIAN_POINT('Origin',(1.23743686707646,-1.23743686707646,2.9));
#9564=CARTESIAN_POINT('',(1.07243686707646,-1.23743686707646,2.9));
#9565=CARTESIAN_POINT('Origin',(1.23743686707646,-1.23743686707646,2.9));
#9566=CARTESIAN_POINT('',(1.07243686707646,-1.23743686707646,3.6));
#9567=CARTESIAN_POINT('',(1.07243686707646,-1.23743686707646,2.9));
#9568=CARTESIAN_POINT('Origin',(1.23743686707646,-1.23743686707646,3.6));
#9569=CARTESIAN_POINT('Origin',(1.23743686707646,-1.23743686707646,2.9));
#9570=CARTESIAN_POINT('Origin',(-1.76776695296637,-1.76776695296637,2.4));
#9571=CARTESIAN_POINT('',(-1.8139637388702,-1.24480341984751,2.4));
#9572=CARTESIAN_POINT('',(-1.24480341984751,-1.81396373887019,2.4));
#9573=CARTESIAN_POINT('Origin',(0.,0.,2.4));
#9574=CARTESIAN_POINT('Origin',(-1.76776695296637,-1.76776695296637,2.4));
#9575=CARTESIAN_POINT('Origin',(-1.76776695296637,-1.76776695296637,1.8));
#9576=CARTESIAN_POINT('',(-1.8139637388702,-1.24480341984751,1.8));
#9577=CARTESIAN_POINT('',(-1.8139637388702,-1.24480341984751,1.8));
#9578=CARTESIAN_POINT('',(-1.24480341984751,-1.81396373887019,1.8));
#9579=CARTESIAN_POINT('Origin',(-1.76776695296637,-1.76776695296637,1.8));
#9580=CARTESIAN_POINT('',(-1.24480341984751,-1.81396373887019,1.8));
#9581=CARTESIAN_POINT('Origin',(-1.76776695296637,1.76776695296637,1.8));
#9582=CARTESIAN_POINT('',(-1.81396373887019,1.24480341984751,2.4));
#9583=CARTESIAN_POINT('',(-1.81396373887019,1.24480341984751,1.8));
#9584=CARTESIAN_POINT('',(-1.81396373887019,1.24480341984751,1.8));
#9585=CARTESIAN_POINT('',(-1.24480341984751,1.81396373887019,2.4));
#9586=CARTESIAN_POINT('Origin',(-1.76776695296637,1.76776695296637,2.4));
#9587=CARTESIAN_POINT('',(-1.24480341984751,1.81396373887019,1.8));
#9588=CARTESIAN_POINT('',(-1.24480341984751,1.81396373887019,1.8));
#9589=CARTESIAN_POINT('Origin',(-1.76776695296637,1.76776695296637,1.8));
#9590=CARTESIAN_POINT('Origin',(-1.76776695296637,1.76776695296637,2.4));
#9591=CARTESIAN_POINT('Origin',(0.,0.,2.4));
#9592=CARTESIAN_POINT('Origin',(1.76776695296637,1.76776695296637,1.8));
#9593=CARTESIAN_POINT('',(1.24480341984751,1.81396373887019,2.4));
#9594=CARTESIAN_POINT('',(1.24480341984751,1.81396373887019,1.8));
#9595=CARTESIAN_POINT('',(1.24480341984751,1.81396373887019,1.8));
#9596=CARTESIAN_POINT('',(1.81396373887019,1.24480341984751,2.4));
#9597=CARTESIAN_POINT('Origin',(1.76776695296637,1.76776695296637,2.4));
#9598=CARTESIAN_POINT('',(1.81396373887019,1.24480341984751,1.8));
#9599=CARTESIAN_POINT('',(1.81396373887019,1.24480341984751,1.8));
#9600=CARTESIAN_POINT('Origin',(1.76776695296637,1.76776695296637,1.8));
#9601=CARTESIAN_POINT('Origin',(1.76776695296637,1.76776695296637,2.4));
#9602=CARTESIAN_POINT('Origin',(0.,0.,2.4));
#9603=CARTESIAN_POINT('Origin',(1.76776695296637,-1.76776695296637,1.8));
#9604=CARTESIAN_POINT('',(1.81396373887019,-1.24480341984751,2.4));
#9605=CARTESIAN_POINT('',(1.81396373887019,-1.24480341984751,1.8));
#9606=CARTESIAN_POINT('',(1.81396373887019,-1.24480341984751,1.8));
#9607=CARTESIAN_POINT('',(1.24480341984751,-1.8139637388702,2.4));
#9608=CARTESIAN_POINT('Origin',(1.76776695296637,-1.76776695296637,2.4));
#9609=CARTESIAN_POINT('',(1.24480341984751,-1.8139637388702,1.8));
#9610=CARTESIAN_POINT('',(1.24480341984751,-1.8139637388702,1.8));
#9611=CARTESIAN_POINT('Origin',(1.76776695296637,-1.76776695296637,1.8));
#9612=CARTESIAN_POINT('Origin',(1.76776695296637,-1.76776695296637,2.4));
#9613=CARTESIAN_POINT('Origin',(0.,0.,2.4));
#9614=CARTESIAN_POINT('Origin',(0.,0.,1.));
#9615=CARTESIAN_POINT('',(-2.2,-2.69422295812418E-16,3.6));
#9616=CARTESIAN_POINT('Origin',(0.,0.,3.6));
#9617=CARTESIAN_POINT('',(-2.2,-2.69422295812418E-16,1.8));
#9618=CARTESIAN_POINT('',(-2.2,-2.69422295812418E-16,1.));
#9619=CARTESIAN_POINT('Origin',(0.,0.,1.8));
#9620=CARTESIAN_POINT('Origin',(0.,0.,1.8));
#9621=CARTESIAN_POINT('Origin',(0.,0.,1.8));
#9622=CARTESIAN_POINT('Origin',(0.,0.,1.8));
#9623=CARTESIAN_POINT('Origin',(0.,0.,1.8));
#9624=CARTESIAN_POINT('Origin',(0.,0.,1.8));
#9625=CARTESIAN_POINT('',(-3.,-3.67394039744206E-16,1.8));
#9626=CARTESIAN_POINT('Origin',(0.,0.,1.8));
#9627=CARTESIAN_POINT('',(-2.04276695296637,-1.76776695296637,1.8));
#9628=CARTESIAN_POINT('Origin',(-1.76776695296637,-1.76776695296637,1.8));
#9629=CARTESIAN_POINT('',(1.49276695296637,1.76776695296637,1.8));
#9630=CARTESIAN_POINT('Origin',(1.76776695296637,1.76776695296637,1.8));
#9631=CARTESIAN_POINT('',(1.49276695296637,-1.76776695296637,1.8));
#9632=CARTESIAN_POINT('Origin',(1.76776695296637,-1.76776695296637,1.8));
#9633=CARTESIAN_POINT('',(-2.04276695296637,1.76776695296637,1.8));
#9634=CARTESIAN_POINT('Origin',(-1.76776695296637,1.76776695296637,1.8));
#9635=CARTESIAN_POINT('Origin',(-1.76776695296637,-1.76776695296637,0.9));
#9636=CARTESIAN_POINT('',(-2.04276695296637,-1.76776695296637,1.));
#9637=CARTESIAN_POINT('Origin',(-1.76776695296637,-1.76776695296637,1.));
#9638=CARTESIAN_POINT('',(-2.04276695296637,-1.76776695296637,0.9));
#9639=CARTESIAN_POINT('Origin',(-1.76776695296637,1.76776695296637,0.9));
#9640=CARTESIAN_POINT('',(-2.04276695296637,1.76776695296637,1.));
#9641=CARTESIAN_POINT('Origin',(-1.76776695296637,1.76776695296637,1.));
#9642=CARTESIAN_POINT('',(-2.04276695296637,1.76776695296637,0.9));
#9643=CARTESIAN_POINT('Origin',(1.76776695296637,1.76776695296637,0.9));
#9644=CARTESIAN_POINT('',(1.49276695296637,1.76776695296637,1.));
#9645=CARTESIAN_POINT('Origin',(1.76776695296637,1.76776695296637,1.));
#9646=CARTESIAN_POINT('',(1.49276695296637,1.76776695296637,0.9));
#9647=CARTESIAN_POINT('Origin',(1.76776695296637,-1.76776695296637,0.9));
#9648=CARTESIAN_POINT('',(1.49276695296637,-1.76776695296637,1.));
#9649=CARTESIAN_POINT('Origin',(1.76776695296637,-1.76776695296637,1.));
#9650=CARTESIAN_POINT('',(1.49276695296637,-1.76776695296637,0.9));
#9651=CARTESIAN_POINT('Origin',(0.,0.,2.05));
#9652=CARTESIAN_POINT('',(-1.5,-1.83697019872103E-16,2.05));
#9653=CARTESIAN_POINT('Origin',(0.,0.,2.05));
#9654=CARTESIAN_POINT('',(-1.5,1.83697019872103E-16,3.6));
#9655=CARTESIAN_POINT('',(-1.5,-1.83697019872103E-16,2.05));
#9656=CARTESIAN_POINT('Origin',(0.,0.,3.6));
#9657=CARTESIAN_POINT('Origin',(0.,0.,2.05));
#9658=CARTESIAN_POINT('',(-1.02,-1.2491397351303E-16,2.05));
#9659=CARTESIAN_POINT('Origin',(0.,0.,2.05));
#9660=CARTESIAN_POINT('Origin',(0.,0.,1.));
#9661=CARTESIAN_POINT('',(-3.,-3.67394039744206E-16,1.));
#9662=CARTESIAN_POINT('',(-3.,-3.67394039744206E-16,1.));
#9663=CARTESIAN_POINT('Origin',(0.,0.,1.));
#9664=CARTESIAN_POINT('Origin',(0.,0.,1.));
#9665=CARTESIAN_POINT('',(-1.02,-1.2491397351303E-16,1.));
#9666=CARTESIAN_POINT('',(-1.02,-1.2491397351303E-16,1.));
#9667=CARTESIAN_POINT('Origin',(0.,0.,1.));
#9668=CARTESIAN_POINT('Origin',(0.,0.,3.6));
#9669=CARTESIAN_POINT('Origin',(0.,0.,1.));
#10977=UNCERTAINTY_MEASURE_WITH_UNIT(LENGTH_MEASURE(0.001),#11036,
'DISTANCE_ACCURACY_VALUE',
'Maximum model space distance between geometric entities at asserted c
onnectivities');
#11002=UNCERTAINTY_MEASURE_WITH_UNIT(LENGTH_MEASURE(0.001),#11036,
'DISTANCE_ACCURACY_VALUE',
'Maximum model space distance between geometric entities at asserted c
onnectivities');
#11010=(
GEOMETRIC_REPRESENTATION_CONTEXT(3)
GLOBAL_UNCERTAINTY_ASSIGNED_CONTEXT((#10977))
GLOBAL_UNIT_ASSIGNED_CONTEXT((#11036,#11038,#11039))
REPRESENTATION_CONTEXT('','3D')
);
#11035=(
GEOMETRIC_REPRESENTATION_CONTEXT(3)
GLOBAL_UNCERTAINTY_ASSIGNED_CONTEXT((#11002))
GLOBAL_UNIT_ASSIGNED_CONTEXT((#11036,#11038,#11039))
REPRESENTATION_CONTEXT('','3D')
);
#11036=(
LENGTH_UNIT()
NAMED_UNIT(*)
SI_UNIT(.CENTI.,.METRE.)
);
#11038=(
NAMED_UNIT(*)
PLANE_ANGLE_UNIT()
SI_UNIT($,.RADIAN.)
);
#11039=(
NAMED_UNIT(*)
SI_UNIT($,.STERADIAN.)
SOLID_ANGLE_UNIT()
);
#11047=SHAPE_DEFINITION_REPRESENTATION(#11079,#11160);
#11079=PRODUCT_DEFINITION_SHAPE('',$,#11193);
#11160=SHAPE_REPRESENTATION('',(#5148),#11010);
#11185=PRODUCT_DEFINITION_CONTEXT('part definition',#11283,'design');
#11193=PRODUCT_DEFINITION('Pivot pedestal','Pivot pedestal',#11225,#11185);
#11225=PRODUCT_DEFINITION_FORMATION('',$,#11292);
#11283=APPLICATION_CONTEXT(
'Core Data for Automotive Mechanical Design Process');
#11284=PRODUCT_CONTEXT('part definition',#11283,'mechanical');
#11292=PRODUCT('Pivot pedestal','Pivot pedestal','Pivot pedestal',(#11284));
#11394=COLOUR_RGB('Off White',0.89,0.88,0.83);
#11395=FILL_AREA_STYLE_COLOUR('',#11394);
#11396=FILL_AREA_STYLE('',(#11395));
#11397=SURFACE_STYLE_FILL_AREA(#11396);
#11398=SURFACE_SIDE_STYLE('',(#11397));
#11399=SURFACE_STYLE_USAGE(.BOTH.,#11398);
#11400=PRESENTATION_STYLE_ASSIGNMENT((#11399));
ENDSEC;
END-ISO-10303-21;
